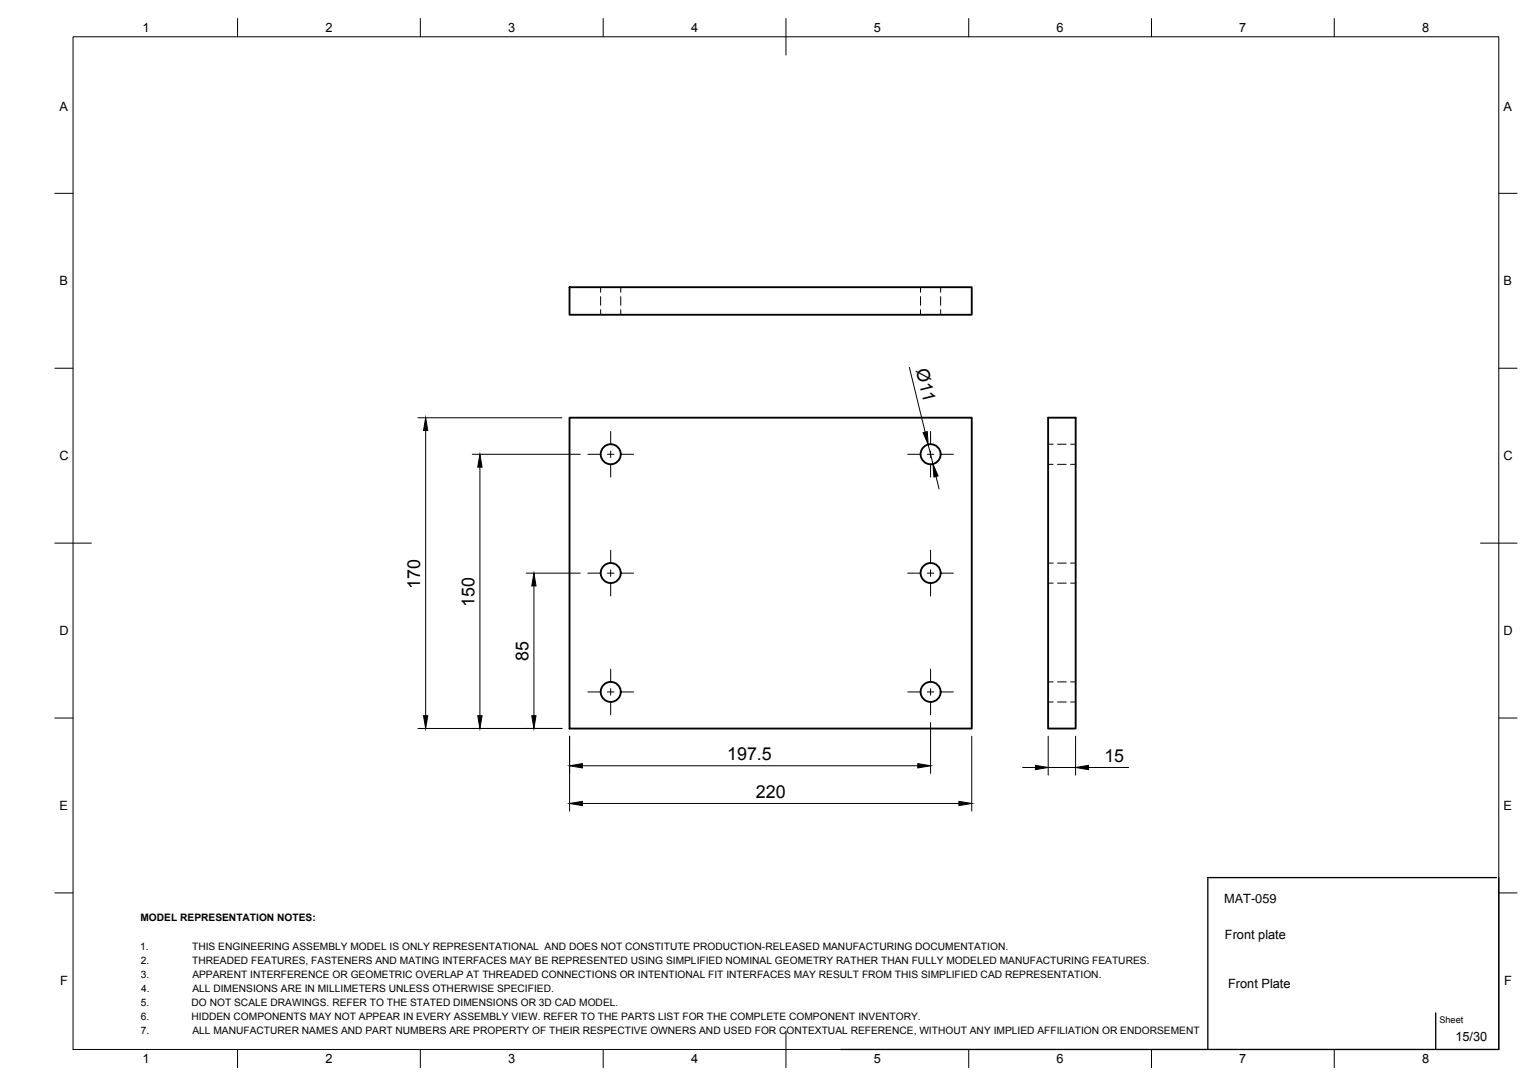
ISO-10303-21;
HEADER;
/* Generated by software containing ST-Developer
 * from STEP Tools, Inc. (www.steptools.com) 
 */

FILE_DESCRIPTION(
/* description */ ('', 'CAx-IF Rec.Pracs.---Representation and Presentation of Product Manufa
cturing Information (PMI)---4.0---2014-10-13'),
/* implementation_level */ '2;1');

FILE_NAME(
/* name */ 'Front Plate.step',
/* time_stamp */ '2026-10-28T23:00:48+01:00',
/* author */ (''),
/* organization */ (''),
/* preprocessor_version */ 'ST-DEVELOPER v20.2',
/* originating_system */ 'Autodesk Translation Framework v15.17.0.0',
/* authorisation */ '');

FILE_SCHEMA (('AP242_MANAGED_MODEL_BASED_3D_ENGINEERING_MIM_LF { 1 0 10303 442 2 1 4 }'));
ENDSEC;

DATA;
#10=MECHANICAL_DESIGN_GEOMETRIC_PRESENTATION_REPRESENTATION('',(#989),#61811);
#925=SHAPE_REPRESENTATION_RELATIONSHIP('SRR','None',#61984,#950);
#950=ADVANCED_BREP_SHAPE_REPRESENTATION('',(#1028),#61797);
#989=STYLED_ITEM('',(#62170),#1028);
#1028=MANIFOLD_SOLID_BREP('Body1',#33819);
#1359=CYLINDRICAL_SURFACE('',#35885,5.5);
#1360=CYLINDRICAL_SURFACE('',#35888,5.5);
#1361=CYLINDRICAL_SURFACE('',#35891,5.5);
#1362=CYLINDRICAL_SURFACE('',#35894,5.5);
#1363=CYLINDRICAL_SURFACE('',#35897,5.5);
#1364=CYLINDRICAL_SURFACE('',#35900,5.5);
#2094=FACE_BOUND('',#7263,.T.);
#2095=FACE_BOUND('',#7264,.T.);
#2096=FACE_BOUND('',#7265,.T.);
#2097=FACE_BOUND('',#7266,.T.);
#2098=FACE_BOUND('',#7267,.T.);
#2099=FACE_BOUND('',#7268,.T.);
#2100=FACE_BOUND('',#7270,.T.);
#2101=FACE_BOUND('',#7271,.T.);
#2102=FACE_BOUND('',#7272,.T.);
#2103=FACE_BOUND('',#7273,.T.);
#2104=FACE_BOUND('',#7274,.T.);
#2105=FACE_BOUND('',#7275,.T.);
#3016=CIRCLE('',#35886,5.5);
#3017=CIRCLE('',#35887,5.5);
#3018=CIRCLE('',#35889,5.5);
#3019=CIRCLE('',#35890,5.5);
#3020=CIRCLE('',#35892,5.5);
#3021=CIRCLE('',#35893,5.5);
#3022=CIRCLE('',#35895,5.5);
#3023=CIRCLE('',#35896,5.5);
#3024=CIRCLE('',#35898,5.5);
#3025=CIRCLE('',#35899,5.5);
#3026=CIRCLE('',#35901,5.5);
#3027=CIRCLE('',#35902,5.5);
#5158=FACE_OUTER_BOUND('',#7252,.T.);
#5159=FACE_OUTER_BOUND('',#7253,.T.);
#5160=FACE_OUTER_BOUND('',#7254,.T.);
#5161=FACE_OUTER_BOUND('',#7255,.T.);
#5162=FACE_OUTER_BOUND('',#7256,.T.);
#5163=FACE_OUTER_BOUND('',#7257,.T.);
#5164=FACE_OUTER_BOUND('',#7258,.T.);
#5165=FACE_OUTER_BOUND('',#7259,.T.);
#5166=FACE_OUTER_BOUND('',#7260,.T.);
#5167=FACE_OUTER_BOUND('',#7261,.T.);
#5168=FACE_OUTER_BOUND('',#7262,.T.);
#5169=FACE_OUTER_BOUND('',#7269,.T.);
#7252=EDGE_LOOP('',(#26062,#26063,#26064,#26065));
#7253=EDGE_LOOP('',(#26066,#26067,#26068,#26069));
#7254=EDGE_LOOP('',(#26070,#26071,#26072,#26073));
#7255=EDGE_LOOP('',(#26074,#26075,#26076,#26077));
#7256=EDGE_LOOP('',(#26078,#26079,#26080,#26081));
#7257=EDGE_LOOP('',(#26082,#26083,#26084,#26085));
#7258=EDGE_LOOP('',(#26086,#26087,#26088,#26089));
#7259=EDGE_LOOP('',(#26090,#26091,#26092,#26093));
#7260=EDGE_LOOP('',(#26094,#26095,#26096,#26097));
#7261=EDGE_LOOP('',(#26098,#26099,#26100,#26101));
#7262=EDGE_LOOP('',(#26102,#26103,#26104,#26105));
#7263=EDGE_LOOP('',(#26106));
#7264=EDGE_LOOP('',(#26107));
#7265=EDGE_LOOP('',(#26108));
#7266=EDGE_LOOP('',(#26109));
#7267=EDGE_LOOP('',(#26110));
#7268=EDGE_LOOP('',(#26111));
#7269=EDGE_LOOP('',(#26112,#26113,#26114,#26115));
#7270=EDGE_LOOP('',(#26116));
#7271=EDGE_LOOP('',(#26117));
#7272=EDGE_LOOP('',(#26118));
#7273=EDGE_LOOP('',(#26119));
#7274=EDGE_LOOP('',(#26120));
#7275=EDGE_LOOP('',(#26121));
#9689=LINE('',#55687,#12236);
#9690=LINE('',#55693,#12237);
#9691=LINE('',#55699,#12238);
#9692=LINE('',#55705,#12239);
#9693=LINE('',#55711,#12240);
#9694=LINE('',#55717,#12241);
#9695=LINE('',#55722,#12242);
#9696=LINE('',#55724,#12243);
#9697=LINE('',#55726,#12244);
#9698=LINE('',#55727,#12245);
#9699=LINE('',#55730,#12246);
#9700=LINE('',#55732,#12247);
#9701=LINE('',#55733,#12248);
#9702=LINE('',#55736,#12249);
#9703=LINE('',#55738,#12250);
#9704=LINE('',#55739,#12251);
#9705=LINE('',#55741,#12252);
#9706=LINE('',#55742,#12253);
#12236=VECTOR('',#43059,5.5);
#12237=VECTOR('',#43066,5.5);
#12238=VECTOR('',#43073,5.5);
#12239=VECTOR('',#43080,5.5);
#12240=VECTOR('',#43087,5.5);
#12241=VECTOR('',#43094,5.5);
#12242=VECTOR('',#43099,10.);
#12243=VECTOR('',#43100,10.);
#12244=VECTOR('',#43101,10.);
#12245=VECTOR('',#43102,10.);
#12246=VECTOR('',#43105,10.);
#12247=VECTOR('',#43106,10.);
#12248=VECTOR('',#43107,10.);
#12249=VECTOR('',#43110,10.);
#12250=VECTOR('',#43111,10.);
#12251=VECTOR('',#43112,10.);
#12252=VECTOR('',#43115,10.);
#12253=VECTOR('',#43116,10.);
#14942=VERTEX_POINT('',#55684);
#14943=VERTEX_POINT('',#55686);
#14944=VERTEX_POINT('',#55690);
#14945=VERTEX_POINT('',#55692);
#14946=VERTEX_POINT('',#55696);
#14947=VERTEX_POINT('',#55698);
#14948=VERTEX_POINT('',#55702);
#14949=VERTEX_POINT('',#55704);
#14950=VERTEX_POINT('',#55708);
#14951=VERTEX_POINT('',#55710);
#14952=VERTEX_POINT('',#55714);
#14953=VERTEX_POINT('',#55716);
#14954=VERTEX_POINT('',#55720);
#14955=VERTEX_POINT('',#55721);
#14956=VERTEX_POINT('',#55723);
#14957=VERTEX_POINT('',#55725);
#14958=VERTEX_POINT('',#55729);
#14959=VERTEX_POINT('',#55731);
#14960=VERTEX_POINT('',#55735);
#14961=VERTEX_POINT('',#55737);
#18933=EDGE_CURVE('',#14942,#14942,#3016,.T.);
#18934=EDGE_CURVE('',#14942,#14943,#9689,.T.);
#18935=EDGE_CURVE('',#14943,#14943,#3017,.T.);
#18936=EDGE_CURVE('',#14944,#14944,#3018,.T.);
#18937=EDGE_CURVE('',#14944,#14945,#9690,.T.);
#18938=EDGE_CURVE('',#14945,#14945,#3019,.T.);
#18939=EDGE_CURVE('',#14946,#14946,#3020,.T.);
#18940=EDGE_CURVE('',#14946,#14947,#9691,.T.);
#18941=EDGE_CURVE('',#14947,#14947,#3021,.T.);
#18942=EDGE_CURVE('',#14948,#14948,#3022,.T.);
#18943=EDGE_CURVE('',#14948,#14949,#9692,.T.);
#18944=EDGE_CURVE('',#14949,#14949,#3023,.T.);
#18945=EDGE_CURVE('',#14950,#14950,#3024,.T.);
#18946=EDGE_CURVE('',#14950,#14951,#9693,.T.);
#18947=EDGE_CURVE('',#14951,#14951,#3025,.T.);
#18948=EDGE_CURVE('',#14952,#14952,#3026,.T.);
#18949=EDGE_CURVE('',#14952,#14953,#9694,.T.);
#18950=EDGE_CURVE('',#14953,#14953,#3027,.T.);
#18951=EDGE_CURVE('',#14954,#14955,#9695,.T.);
#18952=EDGE_CURVE('',#14955,#14956,#9696,.T.);
#18953=EDGE_CURVE('',#14957,#14956,#9697,.T.);
#18954=EDGE_CURVE('',#14954,#14957,#9698,.T.);
#18955=EDGE_CURVE('',#14958,#14954,#9699,.T.);
#18956=EDGE_CURVE('',#14959,#14957,#9700,.T.);
#18957=EDGE_CURVE('',#14958,#14959,#9701,.T.);
#18958=EDGE_CURVE('',#14960,#14958,#9702,.T.);
#18959=EDGE_CURVE('',#14961,#14959,#9703,.T.);
#18960=EDGE_CURVE('',#14960,#14961,#9704,.T.);
#18961=EDGE_CURVE('',#14955,#14960,#9705,.T.);
#18962=EDGE_CURVE('',#14956,#14961,#9706,.T.);
#26062=ORIENTED_EDGE('',*,*,#18933,.F.);
#26063=ORIENTED_EDGE('',*,*,#18934,.T.);
#26064=ORIENTED_EDGE('',*,*,#18935,.F.);
#26065=ORIENTED_EDGE('',*,*,#18934,.F.);
#26066=ORIENTED_EDGE('',*,*,#18936,.F.);
#26067=ORIENTED_EDGE('',*,*,#18937,.T.);
#26068=ORIENTED_EDGE('',*,*,#18938,.F.);
#26069=ORIENTED_EDGE('',*,*,#18937,.F.);
#26070=ORIENTED_EDGE('',*,*,#18939,.F.);
#26071=ORIENTED_EDGE('',*,*,#18940,.T.);
#26072=ORIENTED_EDGE('',*,*,#18941,.F.);
#26073=ORIENTED_EDGE('',*,*,#18940,.F.);
#26074=ORIENTED_EDGE('',*,*,#18942,.F.);
#26075=ORIENTED_EDGE('',*,*,#18943,.T.);
#26076=ORIENTED_EDGE('',*,*,#18944,.F.);
#26077=ORIENTED_EDGE('',*,*,#18943,.F.);
#26078=ORIENTED_EDGE('',*,*,#18945,.F.);
#26079=ORIENTED_EDGE('',*,*,#18946,.T.);
#26080=ORIENTED_EDGE('',*,*,#18947,.F.);
#26081=ORIENTED_EDGE('',*,*,#18946,.F.);
#26082=ORIENTED_EDGE('',*,*,#18948,.F.);
#26083=ORIENTED_EDGE('',*,*,#18949,.T.);
#26084=ORIENTED_EDGE('',*,*,#18950,.F.);
#26085=ORIENTED_EDGE('',*,*,#18949,.F.);
#26086=ORIENTED_EDGE('',*,*,#18951,.T.);
#26087=ORIENTED_EDGE('',*,*,#18952,.T.);
#26088=ORIENTED_EDGE('',*,*,#18953,.F.);
#26089=ORIENTED_EDGE('',*,*,#18954,.F.);
#26090=ORIENTED_EDGE('',*,*,#18955,.T.);
#26091=ORIENTED_EDGE('',*,*,#18954,.T.);
#26092=ORIENTED_EDGE('',*,*,#18956,.F.);
#26093=ORIENTED_EDGE('',*,*,#18957,.F.);
#26094=ORIENTED_EDGE('',*,*,#18958,.T.);
#26095=ORIENTED_EDGE('',*,*,#18957,.T.);
#26096=ORIENTED_EDGE('',*,*,#18959,.F.);
#26097=ORIENTED_EDGE('',*,*,#18960,.F.);
#26098=ORIENTED_EDGE('',*,*,#18961,.T.);
#26099=ORIENTED_EDGE('',*,*,#18960,.T.);
#26100=ORIENTED_EDGE('',*,*,#18962,.F.);
#26101=ORIENTED_EDGE('',*,*,#18952,.F.);
#26102=ORIENTED_EDGE('',*,*,#18962,.T.);
#26103=ORIENTED_EDGE('',*,*,#18959,.T.);
#26104=ORIENTED_EDGE('',*,*,#18956,.T.);
#26105=ORIENTED_EDGE('',*,*,#18953,.T.);
#26106=ORIENTED_EDGE('',*,*,#18935,.T.);
#26107=ORIENTED_EDGE('',*,*,#18938,.T.);
#26108=ORIENTED_EDGE('',*,*,#18941,.T.);
#26109=ORIENTED_EDGE('',*,*,#18944,.T.);
#26110=ORIENTED_EDGE('',*,*,#18947,.T.);
#26111=ORIENTED_EDGE('',*,*,#18950,.T.);
#26112=ORIENTED_EDGE('',*,*,#18961,.F.);
#26113=ORIENTED_EDGE('',*,*,#18951,.F.);
#26114=ORIENTED_EDGE('',*,*,#18955,.F.);
#26115=ORIENTED_EDGE('',*,*,#18958,.F.);
#26116=ORIENTED_EDGE('',*,*,#18933,.T.);
#26117=ORIENTED_EDGE('',*,*,#18936,.T.);
#26118=ORIENTED_EDGE('',*,*,#18939,.T.);
#26119=ORIENTED_EDGE('',*,*,#18942,.T.);
#26120=ORIENTED_EDGE('',*,*,#18945,.T.);
#26121=ORIENTED_EDGE('',*,*,#18948,.T.);
#31600=PLANE('',#35903);
#31601=PLANE('',#35904);
#31602=PLANE('',#35905);
#31603=PLANE('',#35906);
#31604=PLANE('',#35907);
#31605=PLANE('',#35908);
#32839=ADVANCED_FACE('',(#5158),#1359,.F.);
#32840=ADVANCED_FACE('',(#5159),#1360,.F.);
#32841=ADVANCED_FACE('',(#5160),#1361,.F.);
#32842=ADVANCED_FACE('',(#5161),#1362,.F.);
#32843=ADVANCED_FACE('',(#5162),#1363,.F.);
#32844=ADVANCED_FACE('',(#5163),#1364,.F.);
#32845=ADVANCED_FACE('',(#5164),#31600,.T.);
#32846=ADVANCED_FACE('',(#5165),#31601,.T.);
#32847=ADVANCED_FACE('',(#5166),#31602,.T.);
#32848=ADVANCED_FACE('',(#5167),#31603,.T.);
#32849=ADVANCED_FACE('',(#5168,#2094,#2095,#2096,#2097,#2098,#2099),#31604,
 .T.);
#32850=ADVANCED_FACE('',(#5169,#2100,#2101,#2102,#2103,#2104,#2105),#31605,
 .F.);
#33819=CLOSED_SHELL('',(#32839,#32840,#32841,#32842,#32843,#32844,#32845,
#32846,#32847,#32848,#32849,#32850));
#35884=AXIS2_PLACEMENT_3D('',#55682,#43053,#43054);
#35885=AXIS2_PLACEMENT_3D('',#55683,#43055,#43056);
#35886=AXIS2_PLACEMENT_3D('',#55685,#43057,#43058);
#35887=AXIS2_PLACEMENT_3D('',#55688,#43060,#43061);
#35888=AXIS2_PLACEMENT_3D('',#55689,#43062,#43063);
#35889=AXIS2_PLACEMENT_3D('',#55691,#43064,#43065);
#35890=AXIS2_PLACEMENT_3D('',#55694,#43067,#43068);
#35891=AXIS2_PLACEMENT_3D('',#55695,#43069,#43070);
#35892=AXIS2_PLACEMENT_3D('',#55697,#43071,#43072);
#35893=AXIS2_PLACEMENT_3D('',#55700,#43074,#43075);
#35894=AXIS2_PLACEMENT_3D('',#55701,#43076,#43077);
#35895=AXIS2_PLACEMENT_3D('',#55703,#43078,#43079);
#35896=AXIS2_PLACEMENT_3D('',#55706,#43081,#43082);
#35897=AXIS2_PLACEMENT_3D('',#55707,#43083,#43084);
#35898=AXIS2_PLACEMENT_3D('',#55709,#43085,#43086);
#35899=AXIS2_PLACEMENT_3D('',#55712,#43088,#43089);
#35900=AXIS2_PLACEMENT_3D('',#55713,#43090,#43091);
#35901=AXIS2_PLACEMENT_3D('',#55715,#43092,#43093);
#35902=AXIS2_PLACEMENT_3D('',#55718,#43095,#43096);
#35903=AXIS2_PLACEMENT_3D('',#55719,#43097,#43098);
#35904=AXIS2_PLACEMENT_3D('',#55728,#43103,#43104);
#35905=AXIS2_PLACEMENT_3D('',#55734,#43108,#43109);
#35906=AXIS2_PLACEMENT_3D('',#55740,#43113,#43114);
#35907=AXIS2_PLACEMENT_3D('',#55743,#43117,#43118);
#35908=AXIS2_PLACEMENT_3D('',#55744,#43119,#43120);
#43053=DIRECTION('axis',(0.,0.,1.));
#43054=DIRECTION('refdir',(1.,0.,0.));
#43055=DIRECTION('center_axis',(1.,-5.0059604393446E-16,-3.87506992302588E-15));
#43056=DIRECTION('ref_axis',(-3.87506992302588E-15,3.31747701864093E-15,
-1.));
#43057=DIRECTION('center_axis',(1.,-5.0059604393446E-16,-3.87506992302588E-15));
#43058=DIRECTION('ref_axis',(-3.87506992302588E-15,3.31747701864093E-15,
-1.));
#43059=DIRECTION('',(1.,-5.0059604393446E-16,-3.87506992302588E-15));
#43060=DIRECTION('center_axis',(-1.,5.0059604393446E-16,3.87506992302588E-15));
#43061=DIRECTION('ref_axis',(-3.87506992302588E-15,3.31747701864093E-15,
-1.));
#43062=DIRECTION('center_axis',(1.,-5.0059604393446E-16,-3.87506992302588E-15));
#43063=DIRECTION('ref_axis',(-3.87506992302588E-15,3.31747701864093E-15,
-1.));
#43064=DIRECTION('center_axis',(1.,-5.0059604393446E-16,-3.87506992302588E-15));
#43065=DIRECTION('ref_axis',(-3.87506992302588E-15,3.31747701864093E-15,
-1.));
#43066=DIRECTION('',(1.,-5.0059604393446E-16,-3.87506992302588E-15));
#43067=DIRECTION('center_axis',(-1.,5.0059604393446E-16,3.87506992302588E-15));
#43068=DIRECTION('ref_axis',(-3.87506992302588E-15,3.31747701864093E-15,
-1.));
#43069=DIRECTION('center_axis',(1.,-5.0059604393446E-16,-3.87506992302588E-15));
#43070=DIRECTION('ref_axis',(-3.87506992302588E-15,3.31747701864093E-15,
-1.));
#43071=DIRECTION('center_axis',(1.,-5.0059604393446E-16,-3.87506992302588E-15));
#43072=DIRECTION('ref_axis',(-3.87506992302588E-15,3.31747701864093E-15,
-1.));
#43073=DIRECTION('',(1.,-5.0059604393446E-16,-3.87506992302588E-15));
#43074=DIRECTION('center_axis',(-1.,5.0059604393446E-16,3.87506992302588E-15));
#43075=DIRECTION('ref_axis',(-3.87506992302588E-15,3.31747701864093E-15,
-1.));
#43076=DIRECTION('center_axis',(1.,-5.0059604393446E-16,-3.87506992302588E-15));
#43077=DIRECTION('ref_axis',(-3.87506992302588E-15,3.31747701864093E-15,
-1.));
#43078=DIRECTION('center_axis',(1.,-5.0059604393446E-16,-3.87506992302588E-15));
#43079=DIRECTION('ref_axis',(-3.87506992302588E-15,3.31747701864093E-15,
-1.));
#43080=DIRECTION('',(1.,-5.0059604393446E-16,-3.87506992302588E-15));
#43081=DIRECTION('center_axis',(-1.,5.0059604393446E-16,3.87506992302588E-15));
#43082=DIRECTION('ref_axis',(-3.87506992302588E-15,3.31747701864093E-15,
-1.));
#43083=DIRECTION('center_axis',(1.,-5.0059604393446E-16,-3.87506992302588E-15));
#43084=DIRECTION('ref_axis',(-3.87506992302588E-15,3.31747701864093E-15,
-1.));
#43085=DIRECTION('center_axis',(1.,-5.0059604393446E-16,-3.87506992302588E-15));
#43086=DIRECTION('ref_axis',(-3.87506992302588E-15,3.31747701864093E-15,
-1.));
#43087=DIRECTION('',(1.,-5.0059604393446E-16,-3.87506992302588E-15));
#43088=DIRECTION('center_axis',(-1.,5.0059604393446E-16,3.87506992302588E-15));
#43089=DIRECTION('ref_axis',(-3.87506992302588E-15,3.31747701864093E-15,
-1.));
#43090=DIRECTION('center_axis',(1.,-5.0059604393446E-16,-3.87506992302588E-15));
#43091=DIRECTION('ref_axis',(-3.87506992302588E-15,3.31747701864093E-15,
-1.));
#43092=DIRECTION('center_axis',(1.,-5.0059604393446E-16,-3.87506992302588E-15));
#43093=DIRECTION('ref_axis',(-3.87506992302588E-15,3.31747701864093E-15,
-1.));
#43094=DIRECTION('',(1.,-5.0059604393446E-16,-3.87506992302588E-15));
#43095=DIRECTION('center_axis',(-1.,5.0059604393446E-16,3.87506992302588E-15));
#43096=DIRECTION('ref_axis',(-3.87506992302588E-15,3.31747701864093E-15,
-1.));
#43097=DIRECTION('center_axis',(-3.87506992302588E-15,3.64045098944098E-15,
-1.));
#43098=DIRECTION('ref_axis',(5.00596043934474E-16,1.,3.64045098944098E-15));
#43099=DIRECTION('',(5.00596043934474E-16,1.,3.64045098944098E-15));
#43100=DIRECTION('',(1.,-5.0059604393446E-16,-3.87506992302588E-15));
#43101=DIRECTION('',(5.00596043934474E-16,1.,3.64045098944098E-15));
#43102=DIRECTION('',(1.,-5.0059604393446E-16,-3.87506992302588E-15));
#43103=DIRECTION('center_axis',(-5.00596043934474E-16,-1.,-3.52646017621743E-15));
#43104=DIRECTION('ref_axis',(-3.87506992302588E-15,3.52646017621743E-15,
-1.));
#43105=DIRECTION('',(-3.87506992302588E-15,3.52646017621743E-15,-1.));
#43106=DIRECTION('',(-3.87506992302588E-15,3.52646017621743E-15,-1.));
#43107=DIRECTION('',(1.,-5.0059604393446E-16,-3.87506992302588E-15));
#43108=DIRECTION('center_axis',(3.87506992302588E-15,-3.60968124063133E-15,
1.));
#43109=DIRECTION('ref_axis',(-5.00596043934474E-16,-1.,-3.60968124063133E-15));
#43110=DIRECTION('',(-5.00596043934474E-16,-1.,-3.60968124063133E-15));
#43111=DIRECTION('',(-5.00596043934474E-16,-1.,-3.60968124063133E-15));
#43112=DIRECTION('',(1.,-5.0059604393446E-16,-3.87506992302588E-15));
#43113=DIRECTION('center_axis',(5.00596043934474E-16,1.,3.4742143868233E-15));
#43114=DIRECTION('ref_axis',(3.87506992302588E-15,-3.47421438682331E-15,
1.));
#43115=DIRECTION('',(3.87506992302588E-15,-3.47421438682331E-15,1.));
#43116=DIRECTION('',(3.87506992302588E-15,-3.47421438682331E-15,1.));
#43117=DIRECTION('center_axis',(1.,-5.0059604393446E-16,-3.87506992302588E-15));
#43118=DIRECTION('ref_axis',(-3.87506992302588E-15,3.31747701864093E-15,
-1.));
#43119=DIRECTION('center_axis',(1.,-5.0059604393446E-16,-3.87506992302588E-15));
#43120=DIRECTION('ref_axis',(-3.87506992302588E-15,3.31747701864093E-15,
-1.));
#55682=CARTESIAN_POINT('',(0.,0.,0.));
#55683=CARTESIAN_POINT('Origin',(195.682801924451,-267.97200726879,445.000000551899));
#55684=CARTESIAN_POINT('',(459.115917770968,-267.97200726879,450.500000551898));
#55685=CARTESIAN_POINT('Origin',(459.115917770968,-267.97200726879,445.000000551898));
#55686=CARTESIAN_POINT('',(474.115917770968,-267.97200726879,450.500000551898));
#55687=CARTESIAN_POINT('',(195.682801924451,-267.97200726879,450.500000551899));
#55688=CARTESIAN_POINT('Origin',(474.115917770968,-267.97200726879,445.000000551898));
#55689=CARTESIAN_POINT('Origin',(195.682801924451,-92.9720072687897,380.0000005519));
#55690=CARTESIAN_POINT('',(459.115917770968,-92.9720072687899,385.500000551899));
#55691=CARTESIAN_POINT('Origin',(459.115917770968,-92.9720072687899,380.000000551899));
#55692=CARTESIAN_POINT('',(474.115917770968,-92.9720072687899,385.500000551898));
#55693=CARTESIAN_POINT('',(195.682801924451,-92.9720072687898,385.5000005519));
#55694=CARTESIAN_POINT('Origin',(474.115917770968,-92.9720072687899,380.000000551898));
#55695=CARTESIAN_POINT('Origin',(195.682801924451,-92.9720072687902,510.0000005519));
#55696=CARTESIAN_POINT('',(459.115917770968,-92.9720072687903,515.500000551898));
#55697=CARTESIAN_POINT('Origin',(459.115917770968,-92.9720072687903,510.000000551898));
#55698=CARTESIAN_POINT('',(474.115917770969,-92.9720072687903,515.500000551898));
#55699=CARTESIAN_POINT('',(195.682801924451,-92.9720072687902,515.500000551899));
#55700=CARTESIAN_POINT('Origin',(474.115917770968,-92.9720072687903,510.000000551898));
#55701=CARTESIAN_POINT('Origin',(195.682801924451,-92.97200726879,445.000000551899));
#55702=CARTESIAN_POINT('',(459.115917770968,-92.9720072687901,450.500000551898));
#55703=CARTESIAN_POINT('Origin',(459.115917770968,-92.9720072687901,445.000000551898));
#55704=CARTESIAN_POINT('',(474.115917770968,-92.9720072687901,450.500000551898));
#55705=CARTESIAN_POINT('',(195.682801924451,-92.97200726879,450.500000551899));
#55706=CARTESIAN_POINT('Origin',(474.115917770968,-92.9720072687901,445.000000551898));
#55707=CARTESIAN_POINT('Origin',(195.682801924451,-267.97200726879,380.000000551899));
#55708=CARTESIAN_POINT('',(459.115917770968,-267.97200726879,385.500000551898));
#55709=CARTESIAN_POINT('Origin',(459.115917770968,-267.97200726879,380.000000551898));
#55710=CARTESIAN_POINT('',(474.115917770968,-267.97200726879,385.500000551898));
#55711=CARTESIAN_POINT('',(195.682801924451,-267.97200726879,385.500000551899));
#55712=CARTESIAN_POINT('Origin',(474.115917770968,-267.97200726879,380.000000551898));
#55713=CARTESIAN_POINT('Origin',(195.682801924451,-267.97200726879,510.000000551899));
#55714=CARTESIAN_POINT('',(459.115917770968,-267.97200726879,515.500000551898));
#55715=CARTESIAN_POINT('Origin',(459.115917770968,-267.97200726879,510.000000551898));
#55716=CARTESIAN_POINT('',(474.115917770969,-267.97200726879,515.500000551898));
#55717=CARTESIAN_POINT('',(195.682801924451,-267.97200726879,515.500000551899));
#55718=CARTESIAN_POINT('Origin',(474.115917770968,-267.97200726879,510.000000551898));
#55719=CARTESIAN_POINT('Origin',(459.115917770968,-290.47200726879,360.000000551898));
#55720=CARTESIAN_POINT('',(459.115917770968,-290.47200726879,360.000000551898));
#55721=CARTESIAN_POINT('',(459.115917770968,-70.4720072687898,360.000000551899));
#55722=CARTESIAN_POINT('',(459.115917770968,-290.47200726879,360.000000551898));
#55723=CARTESIAN_POINT('',(474.115917770968,-70.4720072687898,360.000000551899));
#55724=CARTESIAN_POINT('',(459.115917770968,-70.4720072687898,360.000000551899));
#55725=CARTESIAN_POINT('',(474.115917770968,-290.47200726879,360.000000551898));
#55726=CARTESIAN_POINT('',(474.115917770968,-290.47200726879,360.000000551898));
#55727=CARTESIAN_POINT('',(459.115917770968,-290.47200726879,360.000000551898));
#55728=CARTESIAN_POINT('Origin',(459.115917770968,-290.47200726879,530.000000551898));
#55729=CARTESIAN_POINT('',(459.115917770968,-290.47200726879,530.000000551898));
#55730=CARTESIAN_POINT('',(459.115917770968,-290.47200726879,530.000000551898));
#55731=CARTESIAN_POINT('',(474.115917770968,-290.47200726879,530.000000551898));
#55732=CARTESIAN_POINT('',(474.115917770968,-290.47200726879,530.000000551898));
#55733=CARTESIAN_POINT('',(459.115917770968,-290.47200726879,530.000000551898));
#55734=CARTESIAN_POINT('Origin',(459.115917770969,-70.4720072687904,530.000000551899));
#55735=CARTESIAN_POINT('',(459.115917770969,-70.4720072687904,530.000000551899));
#55736=CARTESIAN_POINT('',(459.115917770969,-70.4720072687904,530.000000551899));
#55737=CARTESIAN_POINT('',(474.115917770969,-70.4720072687904,530.000000551899));
#55738=CARTESIAN_POINT('',(474.115917770969,-70.4720072687904,530.000000551899));
#55739=CARTESIAN_POINT('',(459.115917770969,-70.4720072687904,530.000000551899));
#55740=CARTESIAN_POINT('Origin',(459.115917770968,-70.4720072687898,360.000000551899));
#55741=CARTESIAN_POINT('',(459.115917770968,-70.4720072687898,360.000000551899));
#55742=CARTESIAN_POINT('',(474.115917770968,-70.4720072687898,360.000000551899));
#55743=CARTESIAN_POINT('Origin',(474.115917770968,-180.47200726879,445.000000551899));
#55744=CARTESIAN_POINT('Origin',(459.115917770968,-180.47200726879,445.000000551899));
#61766=UNCERTAINTY_MEASURE_WITH_UNIT(LENGTH_MEASURE(0.01),#61812,
'DISTANCE_ACCURACY_VALUE',
'Maximum model space distance between geometric entities at asserted c
onnectivities');
#61780=UNCERTAINTY_MEASURE_WITH_UNIT(LENGTH_MEASURE(0.01),#61812,
'DISTANCE_ACCURACY_VALUE',
'Maximum model space distance between geometric entities at asserted c
onnectivities');
#61797=(
GEOMETRIC_REPRESENTATION_CONTEXT(3)
GLOBAL_UNCERTAINTY_ASSIGNED_CONTEXT((#61766))
GLOBAL_UNIT_ASSIGNED_CONTEXT((#61812,#61814,#61815))
REPRESENTATION_CONTEXT('','3D')
);
#61811=(
GEOMETRIC_REPRESENTATION_CONTEXT(3)
GLOBAL_UNCERTAINTY_ASSIGNED_CONTEXT((#61780))
GLOBAL_UNIT_ASSIGNED_CONTEXT((#61812,#61814,#61815))
REPRESENTATION_CONTEXT('','3D')
);
#61812=(
LENGTH_UNIT()
NAMED_UNIT(*)
SI_UNIT(.MILLI.,.METRE.)
);
#61814=(
NAMED_UNIT(*)
PLANE_ANGLE_UNIT()
SI_UNIT($,.RADIAN.)
);
#61815=(
NAMED_UNIT(*)
SI_UNIT($,.STERADIAN.)
SOLID_ANGLE_UNIT()
);
#61832=SHAPE_DEFINITION_REPRESENTATION(#61862,#61984);
#61862=PRODUCT_DEFINITION_SHAPE('',$,#62015);
#61984=SHAPE_REPRESENTATION('',(#35884),#61797);
#61998=PRODUCT_DEFINITION_CONTEXT('part definition',#62090,'design');
#62015=PRODUCT_DEFINITION('Front Plate','Front Plate',#62045,#61998);
#62045=PRODUCT_DEFINITION_FORMATION('',$,#62108);
#62090=APPLICATION_CONTEXT('Managed model based 3d engineering');
#62091=PRODUCT_CONTEXT('part definition',#62090,'mechanical');
#62108=PRODUCT('Front Plate','Front Plate',$,(#62091));
#62164=COLOUR_RGB('Off White',0.89,0.88,0.83);
#62165=FILL_AREA_STYLE_COLOUR('',#62164);
#62166=FILL_AREA_STYLE('',(#62165));
#62167=SURFACE_STYLE_FILL_AREA(#62166);
#62168=SURFACE_SIDE_STYLE('',(#62167));
#62169=SURFACE_STYLE_USAGE(.BOTH.,#62168);
#62170=PRESENTATION_STYLE_ASSIGNMENT((#62169));
ENDSEC;
END-ISO-10303-21;
